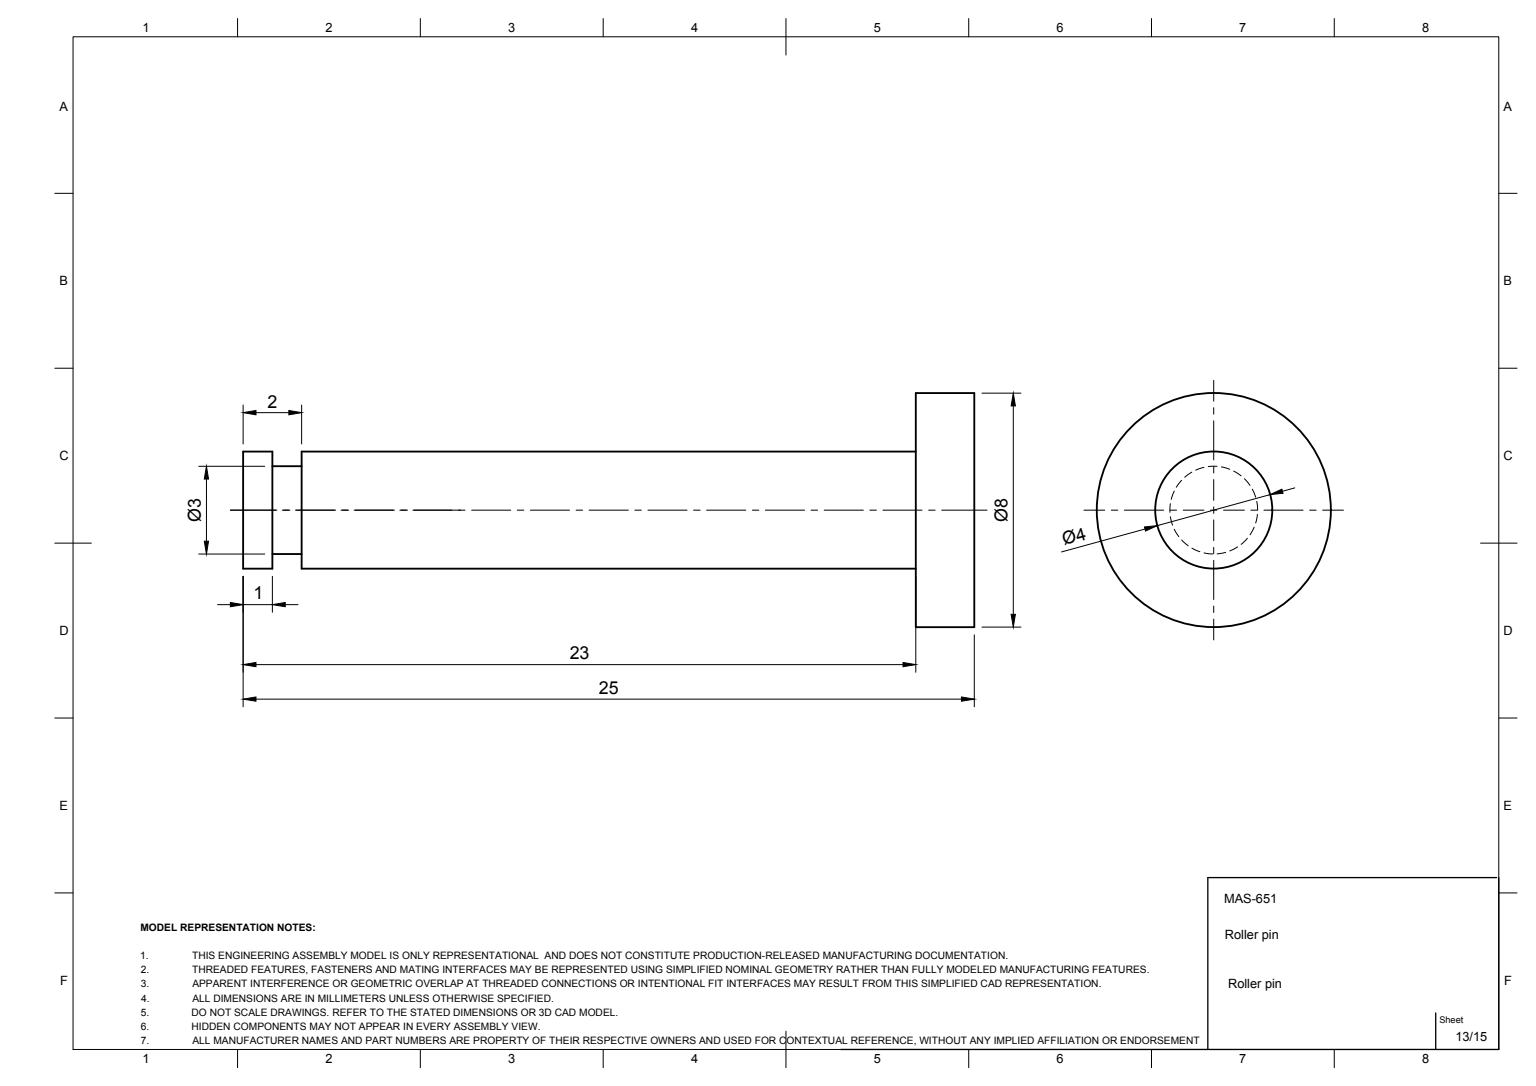
ISO-10303-21;
HEADER;
/* Generated by software containing ST-Developer
 * from STEP Tools, Inc. (www.steptools.com) 
 */

FILE_DESCRIPTION(
/* description */ ('Independent direct-acting normally-closed roller-plunger limit-switch
 CAD. Removable cover, insulated terminal supports, captured bus/conta
ct bridge, native Coil return spring, integral lower travel stop, reus
able instanced hardware and free roller. Manual geometric contact open
ing4mm; no snap-action/contact-force, electrical/current/voltage, envi
ronmental seal, safety-switch, wear, load or life certification. Exter
nal wiring and anchors omitted; fits and application engineering requi
red.'),
/* implementation_level */ '2;1');

FILE_NAME(
/* name */ 'Roller pin.step',
/* time_stamp */ '2026-11-08T07:32:43-08:00',
/* author */ (''),
/* organization */ (''),
/* preprocessor_version */ 'ST-DEVELOPER v20.2',
/* originating_system */ 'Autodesk Translation Framework v15.17.0.0',
/* authorisation */ '');

FILE_SCHEMA (('AUTOMOTIVE_DESIGN { 1 0 10303 214 3 1 1 }'));
ENDSEC;

DATA;
#10=MECHANICAL_DESIGN_GEOMETRIC_PRESENTATION_REPRESENTATION('',(#186),#36482);
#152=SHAPE_REPRESENTATION_RELATIONSHIP('SRR','None',#36565,#169);
#169=ADVANCED_BREP_SHAPE_REPRESENTATION('',(#203),#36475);
#186=STYLED_ITEM('',(#36658),#203);
#203=MANIFOLD_SOLID_BREP('Body1',#9777);
#291=FACE_BOUND('',#1415,.T.);
#292=FACE_BOUND('',#1417,.T.);
#293=FACE_BOUND('',#1420,.T.);
#396=PLANE('',#10466);
#397=PLANE('',#10468);
#398=PLANE('',#10472);
#399=PLANE('',#10477);
#400=PLANE('',#10479);
#819=FACE_OUTER_BOUND('',#1413,.T.);
#820=FACE_OUTER_BOUND('',#1414,.T.);
#821=FACE_OUTER_BOUND('',#1416,.T.);
#822=FACE_OUTER_BOUND('',#1418,.T.);
#823=FACE_OUTER_BOUND('',#1419,.T.);
#824=FACE_OUTER_BOUND('',#1421,.T.);
#825=FACE_OUTER_BOUND('',#1422,.T.);
#826=FACE_OUTER_BOUND('',#1423,.T.);
#827=FACE_OUTER_BOUND('',#1424,.T.);
#1413=EDGE_LOOP('',(#8050,#8051,#8052,#8053));
#1414=EDGE_LOOP('',(#8054));
#1415=EDGE_LOOP('',(#8055));
#1416=EDGE_LOOP('',(#8056));
#1417=EDGE_LOOP('',(#8057));
#1418=EDGE_LOOP('',(#8058,#8059,#8060,#8061));
#1419=EDGE_LOOP('',(#8062));
#1420=EDGE_LOOP('',(#8063));
#1421=EDGE_LOOP('',(#8064,#8065,#8066,#8067));
#1422=EDGE_LOOP('',(#8068));
#1423=EDGE_LOOP('',(#8069,#8070,#8071,#8072));
#1424=EDGE_LOOP('',(#8073));
#1699=CIRCLE('',#10464,0.15);
#1700=CIRCLE('',#10465,0.15);
#1701=CIRCLE('',#10467,0.2);
#1702=CIRCLE('',#10469,0.2);
#1703=CIRCLE('',#10471,0.2);
#1704=CIRCLE('',#10473,0.4);
#1705=CIRCLE('',#10474,0.2);
#1706=CIRCLE('',#10476,0.4);
#2857=LINE('',#29262,#3431);
#2858=LINE('',#29273,#3432);
#2859=LINE('',#29281,#3433);
#2860=LINE('',#29285,#3434);
#3431=VECTOR('',#12088,0.15);
#3432=VECTOR('',#12103,0.2);
#3433=VECTOR('',#12112,0.4);
#3434=VECTOR('',#12119,0.2);
#4279=VERTEX_POINT('',#29259);
#4280=VERTEX_POINT('',#29261);
#4281=VERTEX_POINT('',#29265);
#4282=VERTEX_POINT('',#29268);
#4283=VERTEX_POINT('',#29271);
#4284=VERTEX_POINT('',#29275);
#4285=VERTEX_POINT('',#29277);
#4286=VERTEX_POINT('',#29280);
#5581=EDGE_CURVE('',#4279,#4279,#1699,.T.);
#5582=EDGE_CURVE('',#4279,#4280,#2857,.T.);
#5583=EDGE_CURVE('',#4280,#4280,#1700,.T.);
#5584=EDGE_CURVE('',#4281,#4281,#1701,.T.);
#5585=EDGE_CURVE('',#4282,#4282,#1702,.T.);
#5586=EDGE_CURVE('',#4283,#4283,#1703,.T.);
#5587=EDGE_CURVE('',#4283,#4282,#2858,.T.);
#5588=EDGE_CURVE('',#4284,#4284,#1704,.T.);
#5589=EDGE_CURVE('',#4285,#4285,#1705,.T.);
#5590=EDGE_CURVE('',#4284,#4286,#2859,.T.);
#5591=EDGE_CURVE('',#4286,#4286,#1706,.T.);
#5592=EDGE_CURVE('',#4281,#4285,#2860,.T.);
#8050=ORIENTED_EDGE('',*,*,#5581,.T.);
#8051=ORIENTED_EDGE('',*,*,#5582,.T.);
#8052=ORIENTED_EDGE('',*,*,#5583,.F.);
#8053=ORIENTED_EDGE('',*,*,#5582,.F.);
#8054=ORIENTED_EDGE('',*,*,#5584,.F.);
#8055=ORIENTED_EDGE('',*,*,#5581,.F.);
#8056=ORIENTED_EDGE('',*,*,#5585,.F.);
#8057=ORIENTED_EDGE('',*,*,#5583,.T.);
#8058=ORIENTED_EDGE('',*,*,#5586,.F.);
#8059=ORIENTED_EDGE('',*,*,#5587,.T.);
#8060=ORIENTED_EDGE('',*,*,#5585,.T.);
#8061=ORIENTED_EDGE('',*,*,#5587,.F.);
#8062=ORIENTED_EDGE('',*,*,#5588,.T.);
#8063=ORIENTED_EDGE('',*,*,#5589,.F.);
#8064=ORIENTED_EDGE('',*,*,#5588,.F.);
#8065=ORIENTED_EDGE('',*,*,#5590,.T.);
#8066=ORIENTED_EDGE('',*,*,#5591,.T.);
#8067=ORIENTED_EDGE('',*,*,#5590,.F.);
#8068=ORIENTED_EDGE('',*,*,#5591,.F.);
#8069=ORIENTED_EDGE('',*,*,#5584,.T.);
#8070=ORIENTED_EDGE('',*,*,#5592,.T.);
#8071=ORIENTED_EDGE('',*,*,#5589,.T.);
#8072=ORIENTED_EDGE('',*,*,#5592,.F.);
#8073=ORIENTED_EDGE('',*,*,#5586,.T.);
#9124=CYLINDRICAL_SURFACE('',#10463,0.15);
#9125=CYLINDRICAL_SURFACE('',#10470,0.2);
#9126=CYLINDRICAL_SURFACE('',#10475,0.4);
#9127=CYLINDRICAL_SURFACE('',#10478,0.2);
#9609=ADVANCED_FACE('',(#819),#9124,.T.);
#9610=ADVANCED_FACE('',(#820,#291),#396,.F.);
#9611=ADVANCED_FACE('',(#821,#292),#397,.F.);
#9612=ADVANCED_FACE('',(#822),#9125,.T.);
#9613=ADVANCED_FACE('',(#823,#293),#398,.T.);
#9614=ADVANCED_FACE('',(#824),#9126,.T.);
#9615=ADVANCED_FACE('',(#825),#399,.F.);
#9616=ADVANCED_FACE('',(#826),#9127,.T.);
#9617=ADVANCED_FACE('',(#827),#400,.T.);
#9777=CLOSED_SHELL('',(#9609,#9610,#9611,#9612,#9613,#9614,#9615,#9616,
#9617));
#10462=AXIS2_PLACEMENT_3D('',#29257,#12082,#12083);
#10463=AXIS2_PLACEMENT_3D('',#29258,#12084,#12085);
#10464=AXIS2_PLACEMENT_3D('',#29260,#12086,#12087);
#10465=AXIS2_PLACEMENT_3D('',#29263,#12089,#12090);
#10466=AXIS2_PLACEMENT_3D('',#29264,#12091,#12092);
#10467=AXIS2_PLACEMENT_3D('',#29266,#12093,#12094);
#10468=AXIS2_PLACEMENT_3D('',#29267,#12095,#12096);
#10469=AXIS2_PLACEMENT_3D('',#29269,#12097,#12098);
#10470=AXIS2_PLACEMENT_3D('',#29270,#12099,#12100);
#10471=AXIS2_PLACEMENT_3D('',#29272,#12101,#12102);
#10472=AXIS2_PLACEMENT_3D('',#29274,#12104,#12105);
#10473=AXIS2_PLACEMENT_3D('',#29276,#12106,#12107);
#10474=AXIS2_PLACEMENT_3D('',#29278,#12108,#12109);
#10475=AXIS2_PLACEMENT_3D('',#29279,#12110,#12111);
#10476=AXIS2_PLACEMENT_3D('',#29282,#12113,#12114);
#10477=AXIS2_PLACEMENT_3D('',#29283,#12115,#12116);
#10478=AXIS2_PLACEMENT_3D('',#29284,#12117,#12118);
#10479=AXIS2_PLACEMENT_3D('',#29286,#12120,#12121);
#12082=DIRECTION('axis',(0.,0.,1.));
#12083=DIRECTION('refdir',(1.,0.,0.));
#12084=DIRECTION('center_axis',(0.,0.,1.));
#12085=DIRECTION('ref_axis',(1.,0.,0.));
#12086=DIRECTION('center_axis',(0.,0.,1.));
#12087=DIRECTION('ref_axis',(1.,0.,0.));
#12088=DIRECTION('',(0.,0.,1.));
#12089=DIRECTION('center_axis',(0.,0.,1.));
#12090=DIRECTION('ref_axis',(1.,0.,0.));
#12091=DIRECTION('center_axis',(0.,0.,-1.));
#12092=DIRECTION('ref_axis',(-1.,0.,0.));
#12093=DIRECTION('center_axis',(0.,0.,-1.));
#12094=DIRECTION('ref_axis',(1.,0.,0.));
#12095=DIRECTION('center_axis',(0.,0.,1.));
#12096=DIRECTION('ref_axis',(1.,0.,0.));
#12097=DIRECTION('center_axis',(0.,0.,1.));
#12098=DIRECTION('ref_axis',(1.,0.,0.));
#12099=DIRECTION('center_axis',(0.,0.,1.));
#12100=DIRECTION('ref_axis',(1.,0.,0.));
#12101=DIRECTION('center_axis',(0.,0.,1.));
#12102=DIRECTION('ref_axis',(1.,0.,0.));
#12103=DIRECTION('',(0.,0.,-1.));
#12104=DIRECTION('center_axis',(0.,0.,1.));
#12105=DIRECTION('ref_axis',(1.,0.,0.));
#12106=DIRECTION('center_axis',(0.,0.,1.));
#12107=DIRECTION('ref_axis',(1.,0.,0.));
#12108=DIRECTION('center_axis',(0.,0.,1.));
#12109=DIRECTION('ref_axis',(1.,0.,0.));
#12110=DIRECTION('center_axis',(0.,0.,1.));
#12111=DIRECTION('ref_axis',(1.,0.,0.));
#12112=DIRECTION('',(0.,0.,-1.));
#12113=DIRECTION('center_axis',(0.,0.,1.));
#12114=DIRECTION('ref_axis',(1.,0.,0.));
#12115=DIRECTION('center_axis',(0.,0.,1.));
#12116=DIRECTION('ref_axis',(1.,0.,0.));
#12117=DIRECTION('center_axis',(0.,0.,1.));
#12118=DIRECTION('ref_axis',(1.,0.,0.));
#12119=DIRECTION('',(0.,0.,-1.));
#12120=DIRECTION('center_axis',(0.,0.,1.));
#12121=DIRECTION('ref_axis',(1.,0.,0.));
#29257=CARTESIAN_POINT('',(0.,0.,0.));
#29258=CARTESIAN_POINT('Origin',(0.,0.,2.15));
#29259=CARTESIAN_POINT('',(-0.15,-1.83697019872103E-17,2.1));
#29260=CARTESIAN_POINT('Origin',(0.,0.,2.1));
#29261=CARTESIAN_POINT('',(-0.15,-1.83697019872103E-17,2.2));
#29262=CARTESIAN_POINT('',(-0.15,-1.83697019872103E-17,2.15));
#29263=CARTESIAN_POINT('Origin',(0.,0.,2.2));
#29264=CARTESIAN_POINT('Origin',(0.55,0.,2.1));
#29265=CARTESIAN_POINT('',(-0.2,2.44929359829471E-17,2.1));
#29266=CARTESIAN_POINT('Origin',(0.,0.,2.1));
#29267=CARTESIAN_POINT('Origin',(0.15,0.,2.2));
#29268=CARTESIAN_POINT('',(-0.2,-2.44929359829471E-17,2.2));
#29269=CARTESIAN_POINT('Origin',(0.,0.,2.2));
#29270=CARTESIAN_POINT('Origin',(0.,0.,0.));
#29271=CARTESIAN_POINT('',(-0.2,-2.44929359829471E-17,2.3));
#29272=CARTESIAN_POINT('Origin',(0.,0.,2.3));
#29273=CARTESIAN_POINT('',(-0.2,-2.44929359829471E-17,0.));
#29274=CARTESIAN_POINT('Origin',(0.,0.,0.));
#29275=CARTESIAN_POINT('',(-0.4,-4.89858719658941E-17,0.));
#29276=CARTESIAN_POINT('Origin',(0.,0.,0.));
#29277=CARTESIAN_POINT('',(-0.2,-2.44929359829471E-17,0.));
#29278=CARTESIAN_POINT('Origin',(0.,0.,0.));
#29279=CARTESIAN_POINT('Origin',(0.,0.,-0.2));
#29280=CARTESIAN_POINT('',(-0.4,-4.89858719658941E-17,-0.2));
#29281=CARTESIAN_POINT('',(-0.4,-4.89858719658941E-17,-0.2));
#29282=CARTESIAN_POINT('Origin',(0.,0.,-0.2));
#29283=CARTESIAN_POINT('Origin',(0.,0.,-0.2));
#29284=CARTESIAN_POINT('Origin',(0.,0.,0.));
#29285=CARTESIAN_POINT('',(-0.2,-2.44929359829471E-17,0.));
#29286=CARTESIAN_POINT('Origin',(0.,0.,2.3));
#36456=UNCERTAINTY_MEASURE_WITH_UNIT(LENGTH_MEASURE(0.001),#36483,
'DISTANCE_ACCURACY_VALUE',
'Maximum model space distance between geometric entities at asserted c
onnectivities');
#36463=UNCERTAINTY_MEASURE_WITH_UNIT(LENGTH_MEASURE(0.001),#36483,
'DISTANCE_ACCURACY_VALUE',
'Maximum model space distance between geometric entities at asserted c
onnectivities');
#36475=(
GEOMETRIC_REPRESENTATION_CONTEXT(3)
GLOBAL_UNCERTAINTY_ASSIGNED_CONTEXT((#36456))
GLOBAL_UNIT_ASSIGNED_CONTEXT((#36483,#36485,#36486))
REPRESENTATION_CONTEXT('','3D')
);
#36482=(
GEOMETRIC_REPRESENTATION_CONTEXT(3)
GLOBAL_UNCERTAINTY_ASSIGNED_CONTEXT((#36463))
GLOBAL_UNIT_ASSIGNED_CONTEXT((#36483,#36485,#36486))
REPRESENTATION_CONTEXT('','3D')
);
#36483=(
LENGTH_UNIT()
NAMED_UNIT(*)
SI_UNIT(.CENTI.,.METRE.)
);
#36485=(
NAMED_UNIT(*)
PLANE_ANGLE_UNIT()
SI_UNIT($,.RADIAN.)
);
#36486=(
NAMED_UNIT(*)
SI_UNIT($,.STERADIAN.)
SOLID_ANGLE_UNIT()
);
#36498=SHAPE_DEFINITION_REPRESENTATION(#36516,#36565);
#36516=PRODUCT_DEFINITION_SHAPE('',$,#36584);
#36565=SHAPE_REPRESENTATION('',(#10462),#36475);
#36572=PRODUCT_DEFINITION_CONTEXT('part definition',#36628,'design');
#36584=PRODUCT_DEFINITION('Roller pin','Roller pin',#36602,#36572);
#36602=PRODUCT_DEFINITION_FORMATION('',$,#36641);
#36628=APPLICATION_CONTEXT(
'Core Data for Automotive Mechanical Design Process');
#36629=PRODUCT_CONTEXT('part definition',#36628,'mechanical');
#36641=PRODUCT('Roller pin','Roller pin',$,(#36629));
#36658=PRESENTATION_STYLE_ASSIGNMENT((#36672));
#36672=SURFACE_STYLE_USAGE(.BOTH.,#36686);
#36686=SURFACE_SIDE_STYLE('',(#36700));
#36700=SURFACE_STYLE_FILL_AREA(#36714);
#36714=FILL_AREA_STYLE('Pin gray',(#36728));
#36728=FILL_AREA_STYLE_COLOUR('Pin gray',#36742);
#36742=COLOUR_RGB('Pin gray',0.576470588235294,0.615686274509804,0.666666666666667);
ENDSEC;
END-ISO-10303-21;
